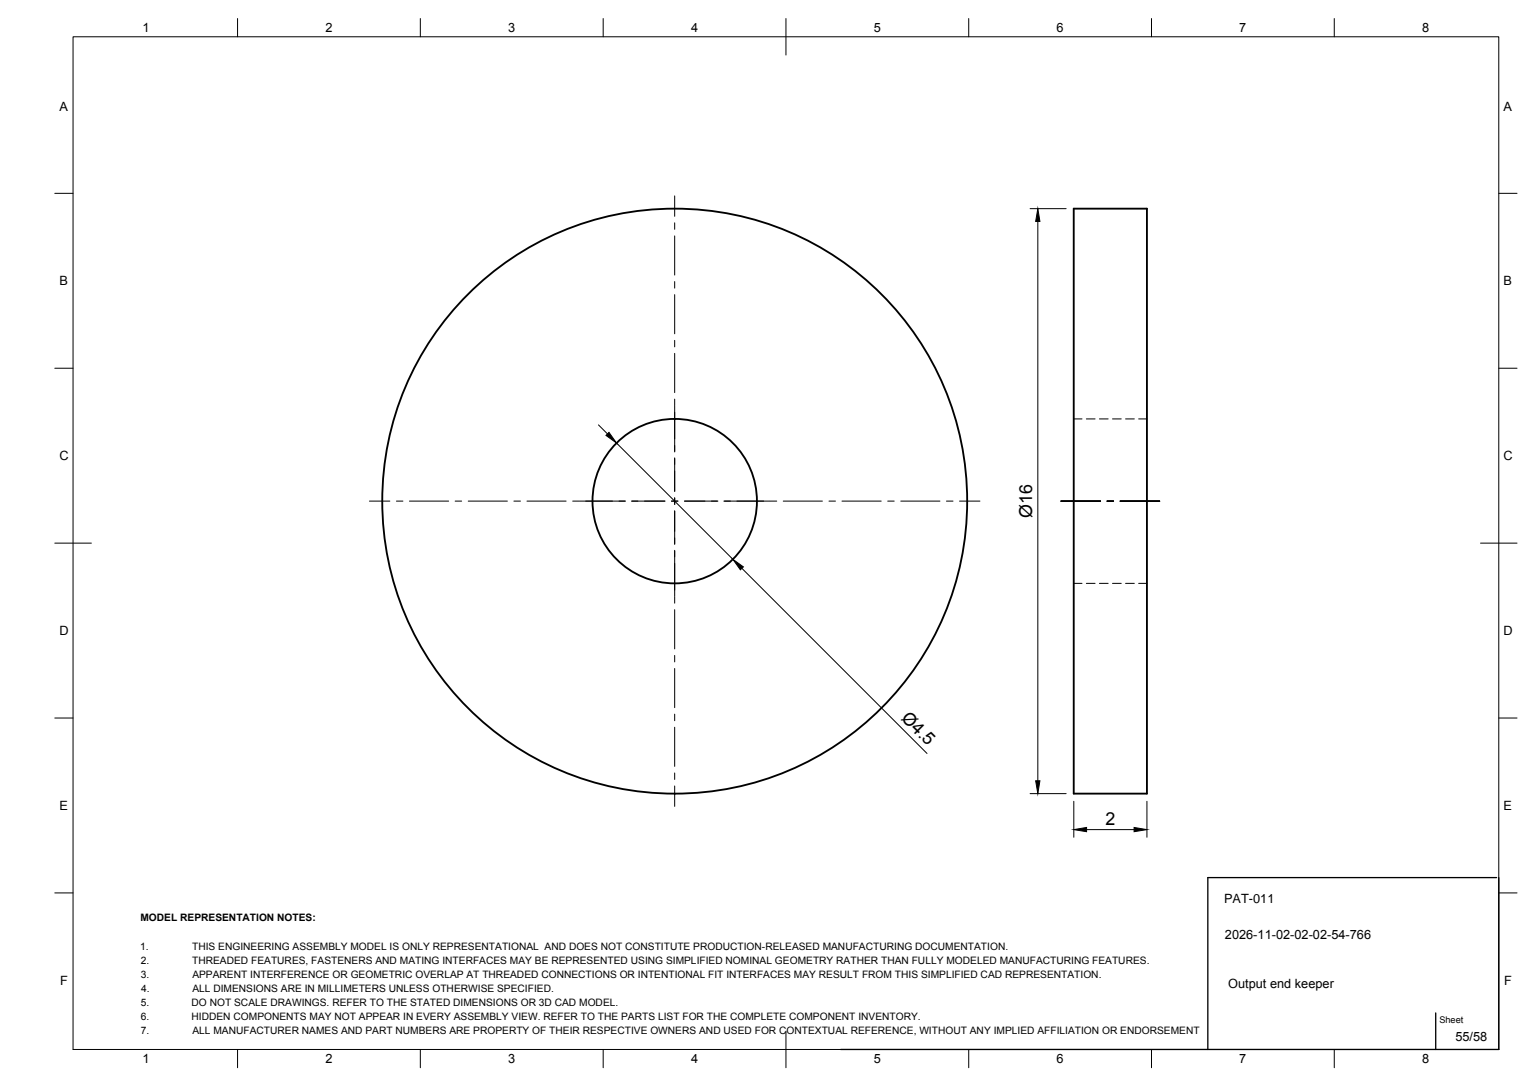
ISO-10303-21;
HEADER;
/* Generated by software containing ST-Developer
 * from STEP Tools, Inc. (www.steptools.com) 
 */

FILE_DESCRIPTION(
/* description */ ('Belt tension measurement rig'),
/* implementation_level */ '2;1');

FILE_NAME(
/* name */ 'Output end keeper.step',
/* time_stamp */ '2026-10-28T03:24:44-07:00',
/* author */ (''),
/* organization */ (''),
/* preprocessor_version */ 'ST-DEVELOPER v20.2',
/* originating_system */ 'Autodesk Translation Framework v15.17.0.0',
/* authorisation */ '');

FILE_SCHEMA (('AUTOMOTIVE_DESIGN { 1 0 10303 214 3 1 1 }'));
ENDSEC;

DATA;
#10=MECHANICAL_DESIGN_GEOMETRIC_PRESENTATION_REPRESENTATION('',(#756),#23587);
#631=SHAPE_REPRESENTATION_RELATIONSHIP('SRR','None',#23882,#686);
#686=ADVANCED_BREP_SHAPE_REPRESENTATION('',(#824),#23580);
#756=STYLED_ITEM('',(#24225),#824);
#824=MANIFOLD_SOLID_BREP('Body1',#12263);
#1013=FACE_BOUND('',#2797,.T.);
#1014=FACE_BOUND('',#2799,.T.);
#1312=PLANE('',#14069);
#1313=PLANE('',#14070);
#1906=FACE_OUTER_BOUND('',#2794,.T.);
#1907=FACE_OUTER_BOUND('',#2795,.T.);
#1908=FACE_OUTER_BOUND('',#2796,.T.);
#1909=FACE_OUTER_BOUND('',#2798,.T.);
#2794=EDGE_LOOP('',(#10384,#10385,#10386,#10387));
#2795=EDGE_LOOP('',(#10388,#10389,#10390,#10391));
#2796=EDGE_LOOP('',(#10392));
#2797=EDGE_LOOP('',(#10393));
#2798=EDGE_LOOP('',(#10394));
#2799=EDGE_LOOP('',(#10395));
#3567=LINE('',#22235,#4318);
#3568=LINE('',#22241,#4319);
#4318=VECTOR('',#17494,0.225);
#4319=VECTOR('',#17501,0.800000000000001);
#5032=CIRCLE('',#14064,0.225);
#5033=CIRCLE('',#14065,0.225);
#5034=CIRCLE('',#14067,0.800000000000001);
#5035=CIRCLE('',#14068,0.800000000000001);
#6069=VERTEX_POINT('',#22232);
#6070=VERTEX_POINT('',#22234);
#6071=VERTEX_POINT('',#22238);
#6072=VERTEX_POINT('',#22240);
#7551=EDGE_CURVE('',#6069,#6069,#5032,.T.);
#7552=EDGE_CURVE('',#6069,#6070,#3567,.T.);
#7553=EDGE_CURVE('',#6070,#6070,#5033,.T.);
#7554=EDGE_CURVE('',#6071,#6071,#5034,.T.);
#7555=EDGE_CURVE('',#6071,#6072,#3568,.T.);
#7556=EDGE_CURVE('',#6072,#6072,#5035,.T.);
#10384=ORIENTED_EDGE('',*,*,#7551,.F.);
#10385=ORIENTED_EDGE('',*,*,#7552,.T.);
#10386=ORIENTED_EDGE('',*,*,#7553,.T.);
#10387=ORIENTED_EDGE('',*,*,#7552,.F.);
#10388=ORIENTED_EDGE('',*,*,#7554,.F.);
#10389=ORIENTED_EDGE('',*,*,#7555,.T.);
#10390=ORIENTED_EDGE('',*,*,#7556,.T.);
#10391=ORIENTED_EDGE('',*,*,#7555,.F.);
#10392=ORIENTED_EDGE('',*,*,#7554,.T.);
#10393=ORIENTED_EDGE('',*,*,#7551,.T.);
#10394=ORIENTED_EDGE('',*,*,#7556,.F.);
#10395=ORIENTED_EDGE('',*,*,#7553,.F.);
#11389=CYLINDRICAL_SURFACE('',#14063,0.225);
#11390=CYLINDRICAL_SURFACE('',#14066,0.800000000000001);
#12047=ADVANCED_FACE('',(#1906),#11389,.F.);
#12048=ADVANCED_FACE('',(#1907),#11390,.T.);
#12049=ADVANCED_FACE('',(#1908,#1013),#1312,.T.);
#12050=ADVANCED_FACE('',(#1909,#1014),#1313,.F.);
#12263=CLOSED_SHELL('',(#12047,#12048,#12049,#12050));
#14062=AXIS2_PLACEMENT_3D('',#22230,#17488,#17489);
#14063=AXIS2_PLACEMENT_3D('',#22231,#17490,#17491);
#14064=AXIS2_PLACEMENT_3D('',#22233,#17492,#17493);
#14065=AXIS2_PLACEMENT_3D('',#22236,#17495,#17496);
#14066=AXIS2_PLACEMENT_3D('',#22237,#17497,#17498);
#14067=AXIS2_PLACEMENT_3D('',#22239,#17499,#17500);
#14068=AXIS2_PLACEMENT_3D('',#22242,#17502,#17503);
#14069=AXIS2_PLACEMENT_3D('',#22243,#17504,#17505);
#14070=AXIS2_PLACEMENT_3D('',#22244,#17506,#17507);
#17488=DIRECTION('axis',(0.,0.,1.));
#17489=DIRECTION('refdir',(1.,0.,0.));
#17490=DIRECTION('center_axis',(0.,1.,0.));
#17491=DIRECTION('ref_axis',(1.,0.,0.));
#17492=DIRECTION('center_axis',(0.,-1.,0.));
#17493=DIRECTION('ref_axis',(1.,0.,0.));
#17494=DIRECTION('',(0.,-1.,0.));
#17495=DIRECTION('center_axis',(0.,-1.,0.));
#17496=DIRECTION('ref_axis',(1.,0.,0.));
#17497=DIRECTION('center_axis',(0.,1.,0.));
#17498=DIRECTION('ref_axis',(1.,0.,0.));
#17499=DIRECTION('center_axis',(0.,1.,0.));
#17500=DIRECTION('ref_axis',(1.,0.,0.));
#17501=DIRECTION('',(0.,-1.,0.));
#17502=DIRECTION('center_axis',(0.,1.,0.));
#17503=DIRECTION('ref_axis',(1.,0.,0.));
#17504=DIRECTION('center_axis',(0.,1.,0.));
#17505=DIRECTION('ref_axis',(1.,0.,0.));
#17506=DIRECTION('center_axis',(0.,1.,0.));
#17507=DIRECTION('ref_axis',(1.,0.,0.));
#22230=CARTESIAN_POINT('',(0.,0.,0.));
#22231=CARTESIAN_POINT('Origin',(10.,-5.2,7.));
#22232=CARTESIAN_POINT('',(9.775,-5.,7.));
#22233=CARTESIAN_POINT('Origin',(10.,-5.,7.));
#22234=CARTESIAN_POINT('',(9.775,-5.2,7.));
#22235=CARTESIAN_POINT('',(9.775,-5.2,7.));
#22236=CARTESIAN_POINT('Origin',(10.,-5.2,7.));
#22237=CARTESIAN_POINT('Origin',(10.,-5.2,7.));
#22238=CARTESIAN_POINT('',(9.2,-5.,7.));
#22239=CARTESIAN_POINT('Origin',(10.,-5.,7.));
#22240=CARTESIAN_POINT('',(9.2,-5.2,7.));
#22241=CARTESIAN_POINT('',(9.2,-5.2,7.));
#22242=CARTESIAN_POINT('Origin',(10.,-5.2,7.));
#22243=CARTESIAN_POINT('Origin',(10.,-5.,7.));
#22244=CARTESIAN_POINT('Origin',(10.,-5.2,7.));
#23515=UNCERTAINTY_MEASURE_WITH_UNIT(LENGTH_MEASURE(0.001),#23588,
'DISTANCE_ACCURACY_VALUE',
'Maximum model space distance between geometric entities at asserted c
onnectivities');
#23522=UNCERTAINTY_MEASURE_WITH_UNIT(LENGTH_MEASURE(0.001),#23588,
'DISTANCE_ACCURACY_VALUE',
'Maximum model space distance between geometric entities at asserted c
onnectivities');
#23580=(
GEOMETRIC_REPRESENTATION_CONTEXT(3)
GLOBAL_UNCERTAINTY_ASSIGNED_CONTEXT((#23515))
GLOBAL_UNIT_ASSIGNED_CONTEXT((#23588,#23590,#23591))
REPRESENTATION_CONTEXT('','3D')
);
#23587=(
GEOMETRIC_REPRESENTATION_CONTEXT(3)
GLOBAL_UNCERTAINTY_ASSIGNED_CONTEXT((#23522))
GLOBAL_UNIT_ASSIGNED_CONTEXT((#23588,#23590,#23591))
REPRESENTATION_CONTEXT('','3D')
);
#23588=(
LENGTH_UNIT()
NAMED_UNIT(*)
SI_UNIT(.CENTI.,.METRE.)
);
#23590=(
NAMED_UNIT(*)
PLANE_ANGLE_UNIT()
SI_UNIT($,.RADIAN.)
);
#23591=(
NAMED_UNIT(*)
SI_UNIT($,.STERADIAN.)
SOLID_ANGLE_UNIT()
);
#23649=SHAPE_DEFINITION_REPRESENTATION(#23726,#23882);
#23726=PRODUCT_DEFINITION_SHAPE('',$,#23947);
#23882=SHAPE_REPRESENTATION('',(#14062),#23580);
#23889=PRODUCT_DEFINITION_CONTEXT('part definition',#24083,'design');
#23947=PRODUCT_DEFINITION('Output end keeper','Output end keeper',#24011,
#23889);
#24011=PRODUCT_DEFINITION_FORMATION('',$,#24142);
#24083=APPLICATION_CONTEXT(
'Core Data for Automotive Mechanical Design Process');
#24084=PRODUCT_CONTEXT('part definition',#24083,'mechanical');
#24142=PRODUCT('Output end keeper','Output end keeper',
'Output end keeper',(#24084));
#24219=COLOUR_RGB('Off White',0.89,0.88,0.83);
#24220=FILL_AREA_STYLE_COLOUR('',#24219);
#24221=FILL_AREA_STYLE('',(#24220));
#24222=SURFACE_STYLE_FILL_AREA(#24221);
#24223=SURFACE_SIDE_STYLE('',(#24222));
#24224=SURFACE_STYLE_USAGE(.BOTH.,#24223);
#24225=PRESENTATION_STYLE_ASSIGNMENT((#24224));
ENDSEC;
END-ISO-10303-21;
